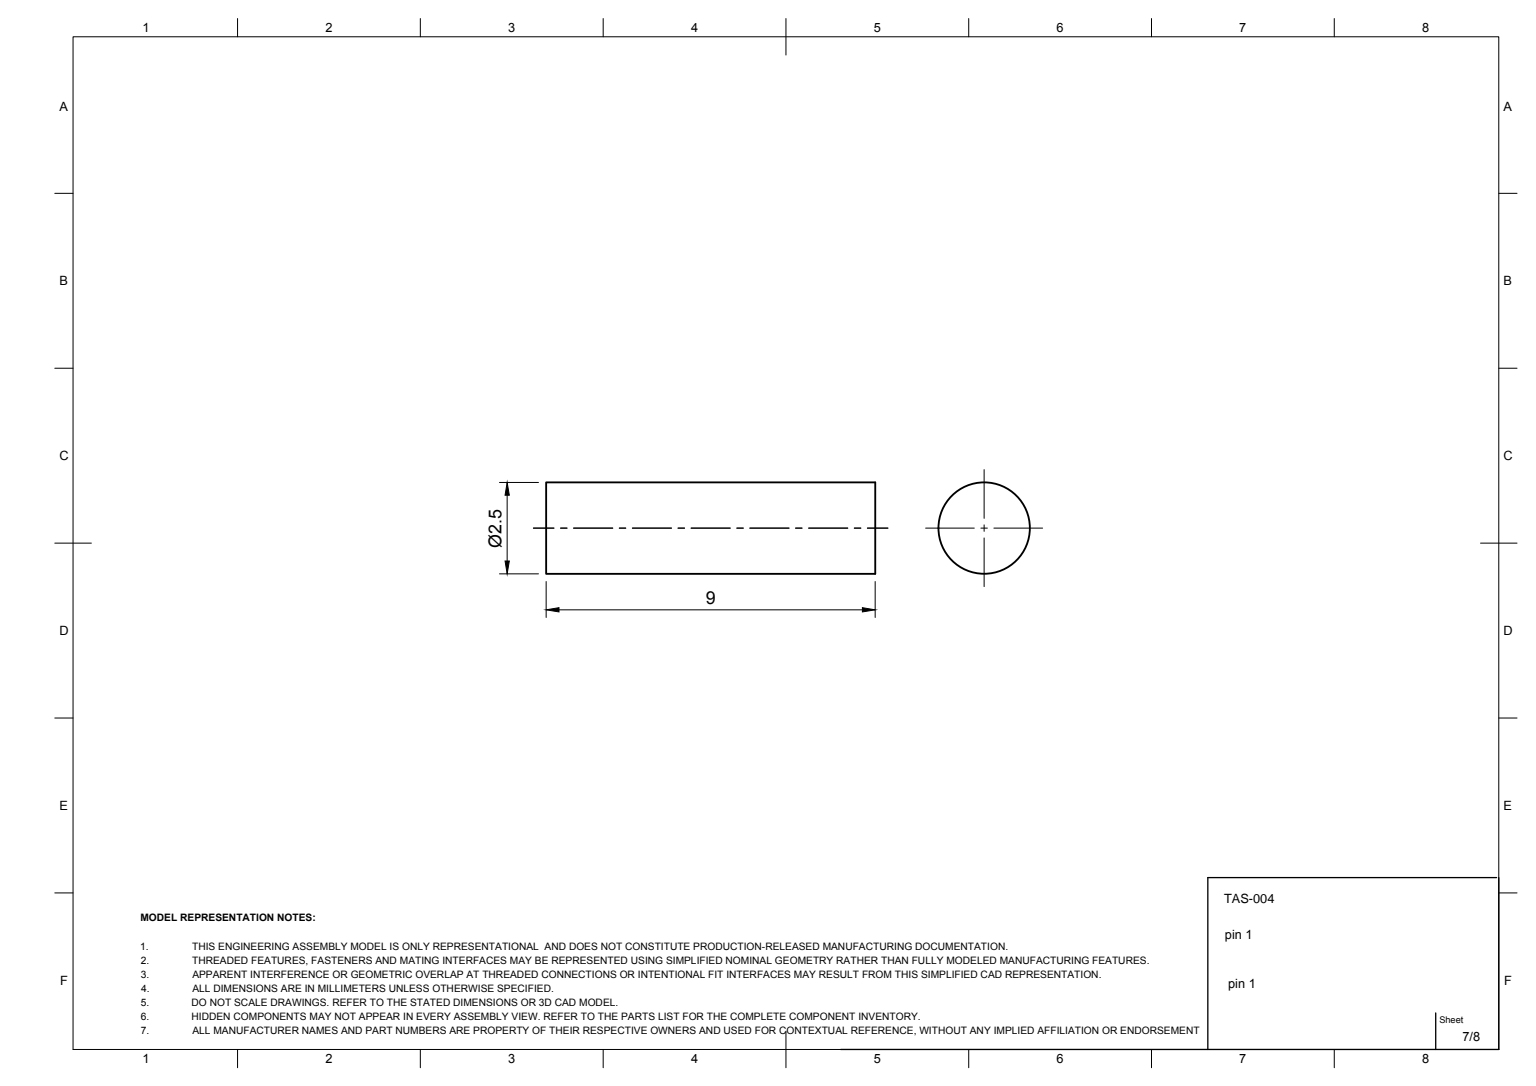
ISO-10303-21;
HEADER;
/* Generated by software containing ST-Developer
 * from STEP Tools, Inc. (www.steptools.com) 
 */

FILE_DESCRIPTION(
/* description */ ('STEP AP214'),
/* implementation_level */ '2;1');

FILE_NAME(
/* name */ 'pin 1.step',
/* time_stamp */ '2026-11-04T19:48:07-08:00',
/* author */ (''),
/* organization */ (''),
/* preprocessor_version */ 'ST-DEVELOPER v20.2',
/* originating_system */ 'Autodesk Translation Framework v15.17.0.0',
/* authorisation */ '');

FILE_SCHEMA (('AUTOMOTIVE_DESIGN { 1 0 10303 214 3 1 1 }'));
ENDSEC;

DATA;
#10=MECHANICAL_DESIGN_GEOMETRIC_PRESENTATION_REPRESENTATION('',(#63),#9561);
#51=SHAPE_REPRESENTATION_RELATIONSHIP('SRR','None',#9591,#57);
#57=ADVANCED_BREP_SHAPE_REPRESENTATION('',(#69),#9559);
#63=STYLED_ITEM('',(#9629),#69);
#69=MANIFOLD_SOLID_BREP('Body1',#2409);
#190=PLANE('',#2682);
#191=PLANE('',#2683);
#331=FACE_OUTER_BOUND('',#489,.T.);
#332=FACE_OUTER_BOUND('',#490,.T.);
#333=FACE_OUTER_BOUND('',#491,.T.);
#489=EDGE_LOOP('',(#2219,#2220,#2221,#2222));
#490=EDGE_LOOP('',(#2223));
#491=EDGE_LOOP('',(#2224));
#743=LINE('',#9527,#993);
#993=VECTOR('',#3350,1.25);
#1057=CIRCLE('',#2680,1.25);
#1058=CIRCLE('',#2681,1.25);
#1255=VERTEX_POINT('',#9524);
#1256=VERTEX_POINT('',#9526);
#1577=EDGE_CURVE('',#1255,#1255,#1057,.T.);
#1578=EDGE_CURVE('',#1255,#1256,#743,.T.);
#1579=EDGE_CURVE('',#1256,#1256,#1058,.T.);
#2219=ORIENTED_EDGE('',*,*,#1577,.T.);
#2220=ORIENTED_EDGE('',*,*,#1578,.T.);
#2221=ORIENTED_EDGE('',*,*,#1579,.F.);
#2222=ORIENTED_EDGE('',*,*,#1578,.F.);
#2223=ORIENTED_EDGE('',*,*,#1579,.T.);
#2224=ORIENTED_EDGE('',*,*,#1577,.F.);
#2260=CYLINDRICAL_SURFACE('',#2679,1.25);
#2399=ADVANCED_FACE('',(#331),#2260,.T.);
#2400=ADVANCED_FACE('',(#332),#190,.T.);
#2401=ADVANCED_FACE('',(#333),#191,.F.);
#2409=CLOSED_SHELL('',(#2399,#2400,#2401));
#2678=AXIS2_PLACEMENT_3D('',#9522,#3344,#3345);
#2679=AXIS2_PLACEMENT_3D('',#9523,#3346,#3347);
#2680=AXIS2_PLACEMENT_3D('',#9525,#3348,#3349);
#2681=AXIS2_PLACEMENT_3D('',#9528,#3351,#3352);
#2682=AXIS2_PLACEMENT_3D('',#9529,#3353,#3354);
#2683=AXIS2_PLACEMENT_3D('',#9530,#3355,#3356);
#3344=DIRECTION('axis',(0.,0.,1.));
#3345=DIRECTION('refdir',(1.,0.,0.));
#3346=DIRECTION('center_axis',(0.,0.,-1.));
#3347=DIRECTION('ref_axis',(-1.,0.,0.));
#3348=DIRECTION('center_axis',(0.,0.,1.));
#3349=DIRECTION('ref_axis',(1.,0.,0.));
#3350=DIRECTION('',(0.,0.,1.));
#3351=DIRECTION('center_axis',(0.,0.,1.));
#3352=DIRECTION('ref_axis',(1.,0.,0.));
#3353=DIRECTION('center_axis',(0.,0.,1.));
#3354=DIRECTION('ref_axis',(1.,0.,0.));
#3355=DIRECTION('center_axis',(0.,0.,1.));
#3356=DIRECTION('ref_axis',(1.,0.,0.));
#9522=CARTESIAN_POINT('',(0.,0.,0.));
#9523=CARTESIAN_POINT('Origin',(0.,0.,4.5));
#9524=CARTESIAN_POINT('',(1.25,-1.53080849893419E-16,-4.5));
#9525=CARTESIAN_POINT('Origin',(0.,0.,-4.5));
#9526=CARTESIAN_POINT('',(1.25,-1.53080849893419E-16,4.5));
#9527=CARTESIAN_POINT('',(1.25,-1.53080849893419E-16,4.5));
#9528=CARTESIAN_POINT('Origin',(0.,0.,4.5));
#9529=CARTESIAN_POINT('Origin',(0.,0.,4.5));
#9530=CARTESIAN_POINT('Origin',(0.,0.,-4.5));
#9551=UNCERTAINTY_MEASURE_WITH_UNIT(LENGTH_MEASURE(0.01),#9562,
'DISTANCE_ACCURACY_VALUE',
'Maximum model space distance between geometric entities at asserted c
onnectivities');
#9553=UNCERTAINTY_MEASURE_WITH_UNIT(LENGTH_MEASURE(0.01),#9562,
'DISTANCE_ACCURACY_VALUE',
'Maximum model space distance between geometric entities at asserted c
onnectivities');
#9559=(
GEOMETRIC_REPRESENTATION_CONTEXT(3)
GLOBAL_UNCERTAINTY_ASSIGNED_CONTEXT((#9551))
GLOBAL_UNIT_ASSIGNED_CONTEXT((#9562,#9564,#9565))
REPRESENTATION_CONTEXT('','3D')
);
#9561=(
GEOMETRIC_REPRESENTATION_CONTEXT(3)
GLOBAL_UNCERTAINTY_ASSIGNED_CONTEXT((#9553))
GLOBAL_UNIT_ASSIGNED_CONTEXT((#9562,#9564,#9565))
REPRESENTATION_CONTEXT('','3D')
);
#9562=(
LENGTH_UNIT()
NAMED_UNIT(*)
SI_UNIT(.MILLI.,.METRE.)
);
#9564=(
NAMED_UNIT(*)
PLANE_ANGLE_UNIT()
SI_UNIT($,.RADIAN.)
);
#9565=(
NAMED_UNIT(*)
SI_UNIT($,.STERADIAN.)
SOLID_ANGLE_UNIT()
);
#9571=SHAPE_DEFINITION_REPRESENTATION(#9578,#9591);
#9578=PRODUCT_DEFINITION_SHAPE('',$,#9599);
#9591=SHAPE_REPRESENTATION('',(#2678),#9559);
#9593=PRODUCT_DEFINITION_CONTEXT('part definition',#9616,'design');
#9599=PRODUCT_DEFINITION('pin 1','pin 1',#9606,#9593);
#9606=PRODUCT_DEFINITION_FORMATION('',$,#9623);
#9616=APPLICATION_CONTEXT(
'Core Data for Automotive Mechanical Design Process');
#9617=PRODUCT_CONTEXT('part definition',#9616,'mechanical');
#9623=PRODUCT('pin 1','pin 1',$,(#9617));
#9629=PRESENTATION_STYLE_ASSIGNMENT((#9634));
#9634=SURFACE_STYLE_USAGE(.BOTH.,#9639);
#9639=SURFACE_SIDE_STYLE('',(#9644));
#9644=SURFACE_STYLE_FILL_AREA(#9649);
#9649=FILL_AREA_STYLE('Opaque(122,133,145)',(#9654));
#9654=FILL_AREA_STYLE_COLOUR('Opaque(122,133,145)',#9659);
#9659=COLOUR_RGB('Opaque(122,133,145)',0.47843137254902,0.52156862745098,
0.568627450980392);
ENDSEC;
END-ISO-10303-21;
